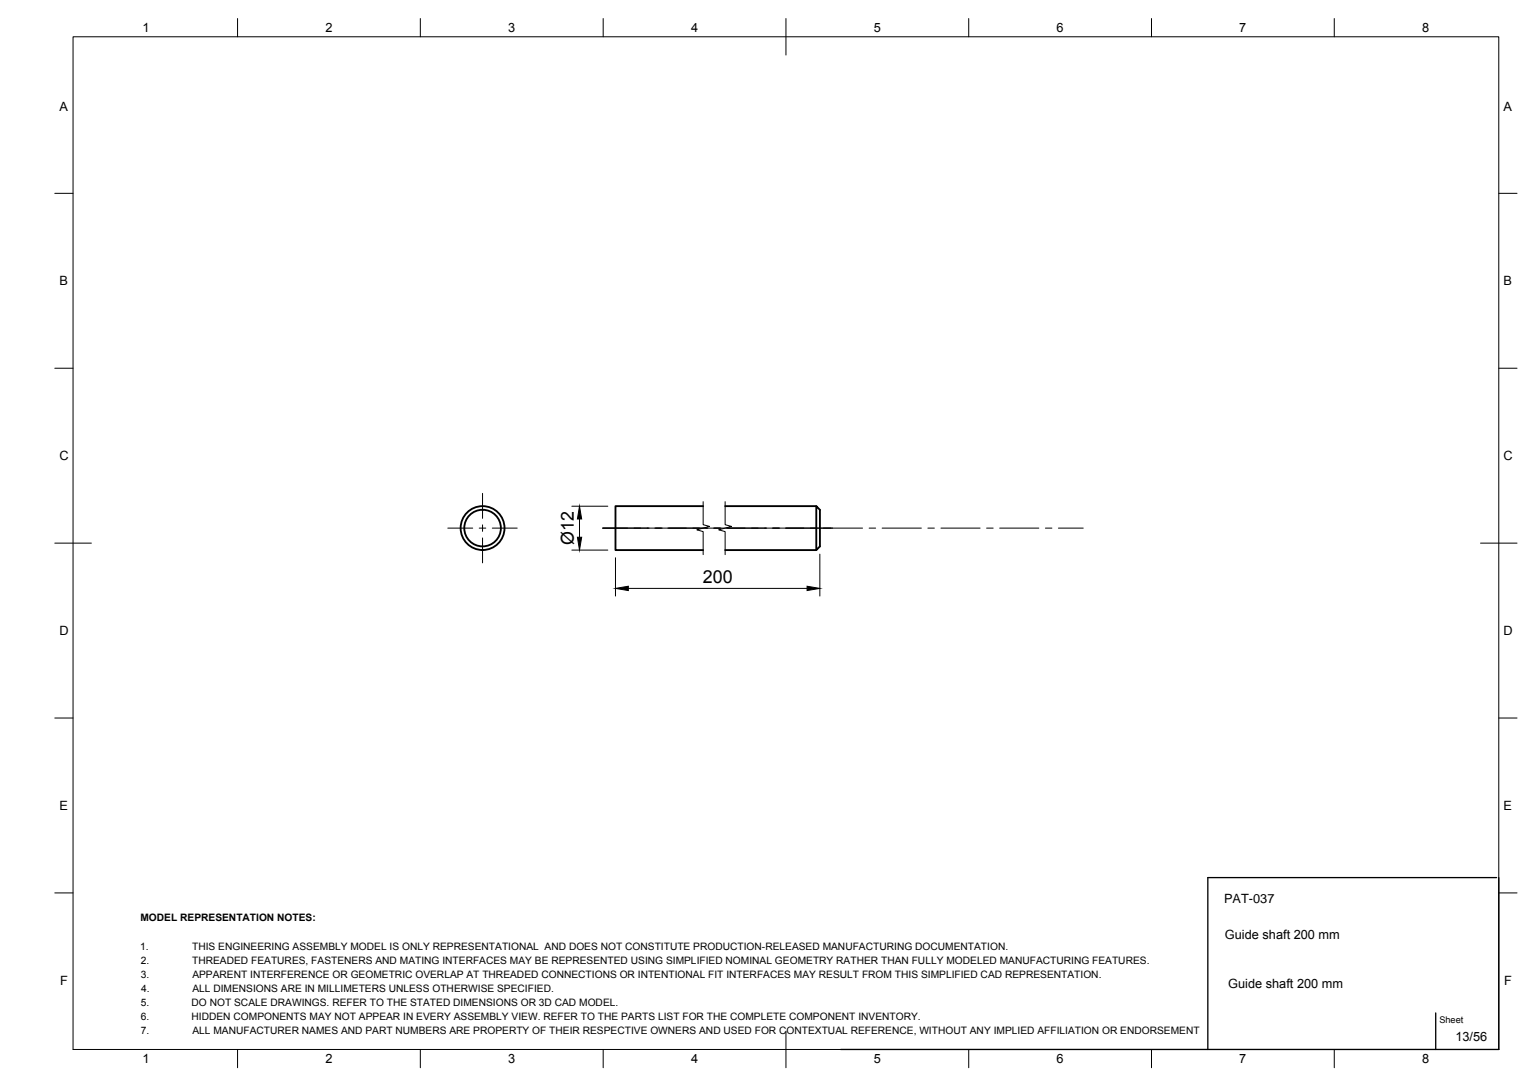
ISO-10303-21;
HEADER;
/* Generated by software containing ST-Developer
 * from STEP Tools, Inc. (www.steptools.com) 
 */

FILE_DESCRIPTION(
/* description */ ('Flywheel Crank-Slider'),
/* implementation_level */ '2;1');

FILE_NAME(
/* name */ 'Guide shaft 200 mm.step',
/* time_stamp */ '2026-10-28T03:23:13-07:00',
/* author */ (''),
/* organization */ (''),
/* preprocessor_version */ 'ST-DEVELOPER v20.2',
/* originating_system */ 'Autodesk Translation Framework v15.17.0.0',
/* authorisation */ '');

FILE_SCHEMA (('AUTOMOTIVE_DESIGN { 1 0 10303 214 3 1 1 }'));
ENDSEC;

DATA;
#10=MECHANICAL_DESIGN_GEOMETRIC_PRESENTATION_REPRESENTATION('',(#689),#17322);
#549=CONICAL_SURFACE('',#10179,0.55,0.785398163397448);
#584=SHAPE_REPRESENTATION_RELATIONSHIP('SRR','None',#17581,#636);
#636=ADVANCED_BREP_SHAPE_REPRESENTATION('',(#746),#17285);
#689=STYLED_ITEM('',(#17931),#746);
#746=MANIFOLD_SOLID_BREP('Body1',#9071);
#1173=PLANE('',#10177);
#1174=PLANE('',#10183);
#1591=FACE_OUTER_BOUND('',#2249,.T.);
#1592=FACE_OUTER_BOUND('',#2250,.T.);
#1593=FACE_OUTER_BOUND('',#2251,.T.);
#1594=FACE_OUTER_BOUND('',#2252,.T.);
#2249=EDGE_LOOP('',(#7268));
#2250=EDGE_LOOP('',(#7269,#7270,#7271,#7272));
#2251=EDGE_LOOP('',(#7273,#7274,#7275,#7276));
#2252=EDGE_LOOP('',(#7277));
#2970=LINE('',#15395,#3581);
#2971=LINE('',#15398,#3582);
#3581=VECTOR('',#12176,0.55);
#3582=VECTOR('',#12181,0.6);
#4033=CIRCLE('',#10178,0.6);
#4034=CIRCLE('',#10180,0.6);
#4035=CIRCLE('',#10181,0.5);
#4656=VERTEX_POINT('',#15389);
#4657=VERTEX_POINT('',#15392);
#4658=VERTEX_POINT('',#15394);
#5591=EDGE_CURVE('',#4656,#4656,#4033,.T.);
#5592=EDGE_CURVE('',#4657,#4657,#4034,.T.);
#5593=EDGE_CURVE('',#4657,#4658,#2970,.T.);
#5594=EDGE_CURVE('',#4658,#4658,#4035,.T.);
#5595=EDGE_CURVE('',#4656,#4657,#2971,.T.);
#7268=ORIENTED_EDGE('',*,*,#5591,.F.);
#7269=ORIENTED_EDGE('',*,*,#5592,.T.);
#7270=ORIENTED_EDGE('',*,*,#5593,.T.);
#7271=ORIENTED_EDGE('',*,*,#5594,.T.);
#7272=ORIENTED_EDGE('',*,*,#5593,.F.);
#7273=ORIENTED_EDGE('',*,*,#5591,.T.);
#7274=ORIENTED_EDGE('',*,*,#5595,.T.);
#7275=ORIENTED_EDGE('',*,*,#5592,.F.);
#7276=ORIENTED_EDGE('',*,*,#5595,.F.);
#7277=ORIENTED_EDGE('',*,*,#5594,.F.);
#8422=CYLINDRICAL_SURFACE('',#10182,0.6);
#8782=ADVANCED_FACE('',(#1591),#1173,.T.);
#8783=ADVANCED_FACE('',(#1592),#549,.T.);
#8784=ADVANCED_FACE('',(#1593),#8422,.T.);
#8785=ADVANCED_FACE('',(#1594),#1174,.F.);
#9071=CLOSED_SHELL('',(#8782,#8783,#8784,#8785));
#10176=AXIS2_PLACEMENT_3D('',#15387,#12166,#12167);
#10177=AXIS2_PLACEMENT_3D('',#15388,#12168,#12169);
#10178=AXIS2_PLACEMENT_3D('',#15390,#12170,#12171);
#10179=AXIS2_PLACEMENT_3D('',#15391,#12172,#12173);
#10180=AXIS2_PLACEMENT_3D('',#15393,#12174,#12175);
#10181=AXIS2_PLACEMENT_3D('',#15396,#12177,#12178);
#10182=AXIS2_PLACEMENT_3D('',#15397,#12179,#12180);
#10183=AXIS2_PLACEMENT_3D('',#15399,#12182,#12183);
#12166=DIRECTION('axis',(0.,0.,1.));
#12167=DIRECTION('refdir',(1.,0.,0.));
#12168=DIRECTION('center_axis',(1.,0.,0.));
#12169=DIRECTION('ref_axis',(0.,0.,-1.));
#12170=DIRECTION('center_axis',(-1.,0.,0.));
#12171=DIRECTION('ref_axis',(0.,0.,-1.));
#12172=DIRECTION('center_axis',(1.,0.,0.));
#12173=DIRECTION('ref_axis',(0.,0.,-1.));
#12174=DIRECTION('center_axis',(-1.,0.,0.));
#12175=DIRECTION('ref_axis',(0.,0.,-1.));
#12176=DIRECTION('',(-0.707106781186548,8.65956056235493E-17,-0.707106781186547));
#12177=DIRECTION('center_axis',(1.,0.,0.));
#12178=DIRECTION('ref_axis',(0.,0.,-1.));
#12179=DIRECTION('center_axis',(1.,0.,0.));
#12180=DIRECTION('ref_axis',(0.,0.,-1.));
#12181=DIRECTION('',(-1.,0.,0.));
#12182=DIRECTION('center_axis',(1.,0.,0.));
#12183=DIRECTION('ref_axis',(0.,0.,-1.));
#15387=CARTESIAN_POINT('',(0.,0.,0.));
#15388=CARTESIAN_POINT('Origin',(20.,0.,0.));
#15389=CARTESIAN_POINT('',(20.,7.34788079488412E-17,0.6));
#15390=CARTESIAN_POINT('Origin',(20.,0.,0.));
#15391=CARTESIAN_POINT('Origin',(0.05,0.,0.));
#15392=CARTESIAN_POINT('',(0.1,7.34788079488412E-17,0.6));
#15393=CARTESIAN_POINT('Origin',(0.1,0.,0.));
#15394=CARTESIAN_POINT('',(0.,-6.12323399573677E-17,0.5));
#15395=CARTESIAN_POINT('',(0.05,-6.73555739531044E-17,0.55));
#15396=CARTESIAN_POINT('Origin',(0.,0.,0.));
#15397=CARTESIAN_POINT('Origin',(0.,0.,0.));
#15398=CARTESIAN_POINT('',(0.,-7.34788079488412E-17,0.6));
#15399=CARTESIAN_POINT('Origin',(0.,0.,0.));
#17224=UNCERTAINTY_MEASURE_WITH_UNIT(LENGTH_MEASURE(0.001),#17323,
'DISTANCE_ACCURACY_VALUE',
'Maximum model space distance between geometric entities at asserted c
onnectivities');
#17261=UNCERTAINTY_MEASURE_WITH_UNIT(LENGTH_MEASURE(0.001),#17323,
'DISTANCE_ACCURACY_VALUE',
'Maximum model space distance between geometric entities at asserted c
onnectivities');
#17285=(
GEOMETRIC_REPRESENTATION_CONTEXT(3)
GLOBAL_UNCERTAINTY_ASSIGNED_CONTEXT((#17224))
GLOBAL_UNIT_ASSIGNED_CONTEXT((#17323,#17325,#17326))
REPRESENTATION_CONTEXT('','3D')
);
#17322=(
GEOMETRIC_REPRESENTATION_CONTEXT(3)
GLOBAL_UNCERTAINTY_ASSIGNED_CONTEXT((#17261))
GLOBAL_UNIT_ASSIGNED_CONTEXT((#17323,#17325,#17326))
REPRESENTATION_CONTEXT('','3D')
);
#17323=(
LENGTH_UNIT()
NAMED_UNIT(*)
SI_UNIT(.CENTI.,.METRE.)
);
#17325=(
NAMED_UNIT(*)
PLANE_ANGLE_UNIT()
SI_UNIT($,.RADIAN.)
);
#17326=(
NAMED_UNIT(*)
SI_UNIT($,.STERADIAN.)
SOLID_ANGLE_UNIT()
);
#17350=SHAPE_DEFINITION_REPRESENTATION(#17412,#17581);
#17412=PRODUCT_DEFINITION_SHAPE('',$,#17642);
#17581=SHAPE_REPRESENTATION('',(#10176),#17285);
#17618=PRODUCT_DEFINITION_CONTEXT('part definition',#17800,'design');
#17642=PRODUCT_DEFINITION('Guide shaft 200 mm','Guide shaft 200 mm',#17702,
#17618);
#17702=PRODUCT_DEFINITION_FORMATION('',$,#17825);
#17800=APPLICATION_CONTEXT(
'Core Data for Automotive Mechanical Design Process');
#17801=PRODUCT_CONTEXT('part definition',#17800,'mechanical');
#17825=PRODUCT('Guide shaft 200 mm','Guide shaft 200 mm',
'Guide shaft 200 mm',(#17801));
#17925=COLOUR_RGB('Grey',0.48,0.52,0.57);
#17926=FILL_AREA_STYLE_COLOUR('',#17925);
#17927=FILL_AREA_STYLE('',(#17926));
#17928=SURFACE_STYLE_FILL_AREA(#17927);
#17929=SURFACE_SIDE_STYLE('',(#17928));
#17930=SURFACE_STYLE_USAGE(.BOTH.,#17929);
#17931=PRESENTATION_STYLE_ASSIGNMENT((#17930));
ENDSEC;
END-ISO-10303-21;
